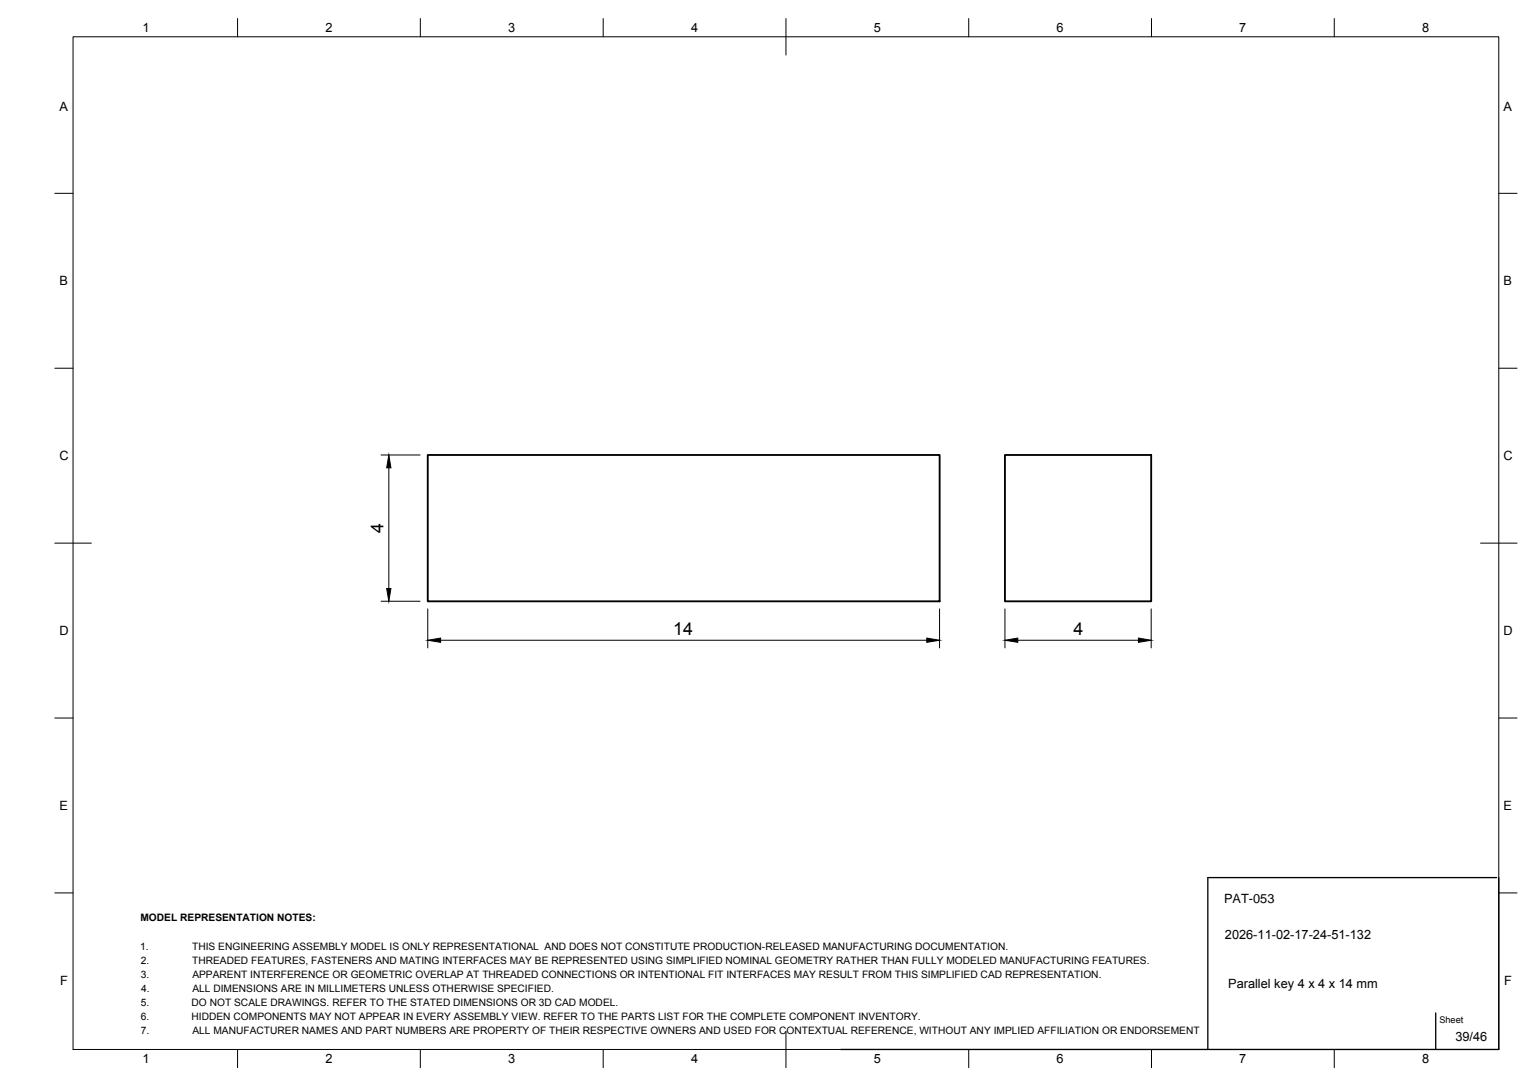
ISO-10303-21;
HEADER;
/* Generated by software containing ST-Developer
 * from STEP Tools, Inc. (www.steptools.com) 
 */

FILE_DESCRIPTION(
/* description */ ('Hand-operated arbor press'),
/* implementation_level */ '2;1');

FILE_NAME(
/* name */ 'Parallel key 4 x 4 x 14 mm.step',
/* time_stamp */ '2026-10-28T03:25:25-07:00',
/* author */ (''),
/* organization */ (''),
/* preprocessor_version */ 'ST-DEVELOPER v20.2',
/* originating_system */ 'Autodesk Translation Framework v15.17.0.0',
/* authorisation */ '');

FILE_SCHEMA (('AUTOMOTIVE_DESIGN { 1 0 10303 214 3 1 1 }'));
ENDSEC;

DATA;
#10=MECHANICAL_DESIGN_GEOMETRIC_PRESENTATION_REPRESENTATION('',(#624),#32751);
#533=SHAPE_REPRESENTATION_RELATIONSHIP('SRR','None',#32965,#575);
#575=ADVANCED_BREP_SHAPE_REPRESENTATION('',(#671),#32739);
#624=STYLED_ITEM('',(#33242),#671);
#671=MANIFOLD_SOLID_BREP('Body1',#12523);
#1214=PLANE('',#13859);
#1215=PLANE('',#13860);
#1216=PLANE('',#13861);
#1217=PLANE('',#13862);
#1218=PLANE('',#13863);
#1219=PLANE('',#13864);
#1807=FACE_OUTER_BOUND('',#2637,.T.);
#1808=FACE_OUTER_BOUND('',#2638,.T.);
#1809=FACE_OUTER_BOUND('',#2639,.T.);
#1810=FACE_OUTER_BOUND('',#2640,.T.);
#1811=FACE_OUTER_BOUND('',#2641,.T.);
#1812=FACE_OUTER_BOUND('',#2642,.T.);
#2637=EDGE_LOOP('',(#10836,#10837,#10838,#10839));
#2638=EDGE_LOOP('',(#10840,#10841,#10842,#10843));
#2639=EDGE_LOOP('',(#10844,#10845,#10846,#10847));
#2640=EDGE_LOOP('',(#10848,#10849,#10850,#10851));
#2641=EDGE_LOOP('',(#10852,#10853,#10854,#10855));
#2642=EDGE_LOOP('',(#10856,#10857,#10858,#10859));
#3762=LINE('',#20662,#4933);
#3763=LINE('',#20664,#4934);
#3764=LINE('',#20666,#4935);
#3765=LINE('',#20667,#4936);
#3766=LINE('',#20670,#4937);
#3767=LINE('',#20672,#4938);
#3768=LINE('',#20673,#4939);
#3769=LINE('',#20676,#4940);
#3770=LINE('',#20678,#4941);
#3771=LINE('',#20679,#4942);
#3772=LINE('',#20681,#4943);
#3773=LINE('',#20682,#4944);
#4933=VECTOR('',#16815,1.);
#4934=VECTOR('',#16816,1.);
#4935=VECTOR('',#16817,1.);
#4936=VECTOR('',#16818,1.);
#4937=VECTOR('',#16821,1.);
#4938=VECTOR('',#16822,1.);
#4939=VECTOR('',#16823,1.);
#4940=VECTOR('',#16826,1.);
#4941=VECTOR('',#16827,1.);
#4942=VECTOR('',#16828,1.);
#4943=VECTOR('',#16831,1.);
#4944=VECTOR('',#16832,1.);
#6399=VERTEX_POINT('',#20660);
#6400=VERTEX_POINT('',#20661);
#6401=VERTEX_POINT('',#20663);
#6402=VERTEX_POINT('',#20665);
#6403=VERTEX_POINT('',#20669);
#6404=VERTEX_POINT('',#20671);
#6405=VERTEX_POINT('',#20675);
#6406=VERTEX_POINT('',#20677);
#7921=EDGE_CURVE('',#6399,#6400,#3762,.T.);
#7922=EDGE_CURVE('',#6400,#6401,#3763,.T.);
#7923=EDGE_CURVE('',#6402,#6401,#3764,.T.);
#7924=EDGE_CURVE('',#6399,#6402,#3765,.T.);
#7925=EDGE_CURVE('',#6403,#6399,#3766,.T.);
#7926=EDGE_CURVE('',#6404,#6402,#3767,.T.);
#7927=EDGE_CURVE('',#6403,#6404,#3768,.T.);
#7928=EDGE_CURVE('',#6405,#6403,#3769,.T.);
#7929=EDGE_CURVE('',#6406,#6404,#3770,.T.);
#7930=EDGE_CURVE('',#6405,#6406,#3771,.T.);
#7931=EDGE_CURVE('',#6400,#6405,#3772,.T.);
#7932=EDGE_CURVE('',#6401,#6406,#3773,.T.);
#10836=ORIENTED_EDGE('',*,*,#7921,.T.);
#10837=ORIENTED_EDGE('',*,*,#7922,.T.);
#10838=ORIENTED_EDGE('',*,*,#7923,.F.);
#10839=ORIENTED_EDGE('',*,*,#7924,.F.);
#10840=ORIENTED_EDGE('',*,*,#7925,.T.);
#10841=ORIENTED_EDGE('',*,*,#7924,.T.);
#10842=ORIENTED_EDGE('',*,*,#7926,.F.);
#10843=ORIENTED_EDGE('',*,*,#7927,.F.);
#10844=ORIENTED_EDGE('',*,*,#7928,.T.);
#10845=ORIENTED_EDGE('',*,*,#7927,.T.);
#10846=ORIENTED_EDGE('',*,*,#7929,.F.);
#10847=ORIENTED_EDGE('',*,*,#7930,.F.);
#10848=ORIENTED_EDGE('',*,*,#7931,.T.);
#10849=ORIENTED_EDGE('',*,*,#7930,.T.);
#10850=ORIENTED_EDGE('',*,*,#7932,.F.);
#10851=ORIENTED_EDGE('',*,*,#7922,.F.);
#10852=ORIENTED_EDGE('',*,*,#7932,.T.);
#10853=ORIENTED_EDGE('',*,*,#7929,.T.);
#10854=ORIENTED_EDGE('',*,*,#7926,.T.);
#10855=ORIENTED_EDGE('',*,*,#7923,.T.);
#10856=ORIENTED_EDGE('',*,*,#7931,.F.);
#10857=ORIENTED_EDGE('',*,*,#7921,.F.);
#10858=ORIENTED_EDGE('',*,*,#7925,.F.);
#10859=ORIENTED_EDGE('',*,*,#7928,.F.);
#12316=ADVANCED_FACE('',(#1807),#1214,.T.);
#12317=ADVANCED_FACE('',(#1808),#1215,.T.);
#12318=ADVANCED_FACE('',(#1809),#1216,.T.);
#12319=ADVANCED_FACE('',(#1810),#1217,.T.);
#12320=ADVANCED_FACE('',(#1811),#1218,.T.);
#12321=ADVANCED_FACE('',(#1812),#1219,.F.);
#12523=CLOSED_SHELL('',(#12316,#12317,#12318,#12319,#12320,#12321));
#13858=AXIS2_PLACEMENT_3D('',#20658,#16811,#16812);
#13859=AXIS2_PLACEMENT_3D('',#20659,#16813,#16814);
#13860=AXIS2_PLACEMENT_3D('',#20668,#16819,#16820);
#13861=AXIS2_PLACEMENT_3D('',#20674,#16824,#16825);
#13862=AXIS2_PLACEMENT_3D('',#20680,#16829,#16830);
#13863=AXIS2_PLACEMENT_3D('',#20683,#16833,#16834);
#13864=AXIS2_PLACEMENT_3D('',#20684,#16835,#16836);
#16811=DIRECTION('axis',(0.,0.,1.));
#16812=DIRECTION('refdir',(1.,0.,0.));
#16813=DIRECTION('center_axis',(0.,1.,0.));
#16814=DIRECTION('ref_axis',(-1.,0.,0.));
#16815=DIRECTION('',(-1.,0.,0.));
#16816=DIRECTION('',(0.,0.,1.));
#16817=DIRECTION('',(-1.,0.,0.));
#16818=DIRECTION('',(0.,0.,1.));
#16819=DIRECTION('center_axis',(1.,0.,0.));
#16820=DIRECTION('ref_axis',(0.,1.,0.));
#16821=DIRECTION('',(0.,1.,0.));
#16822=DIRECTION('',(0.,1.,0.));
#16823=DIRECTION('',(0.,0.,1.));
#16824=DIRECTION('center_axis',(0.,-1.,0.));
#16825=DIRECTION('ref_axis',(1.,0.,0.));
#16826=DIRECTION('',(1.,0.,0.));
#16827=DIRECTION('',(1.,0.,0.));
#16828=DIRECTION('',(0.,0.,1.));
#16829=DIRECTION('center_axis',(-1.,0.,0.));
#16830=DIRECTION('ref_axis',(0.,-1.,0.));
#16831=DIRECTION('',(0.,-1.,0.));
#16832=DIRECTION('',(0.,-1.,0.));
#16833=DIRECTION('center_axis',(0.,0.,1.));
#16834=DIRECTION('ref_axis',(1.,0.,0.));
#16835=DIRECTION('center_axis',(0.,0.,1.));
#16836=DIRECTION('ref_axis',(1.,0.,0.));
#20658=CARTESIAN_POINT('',(0.,0.,0.));
#20659=CARTESIAN_POINT('Origin',(-2.5,1.2,19.8));
#20660=CARTESIAN_POINT('',(-2.5,1.2,19.8));
#20661=CARTESIAN_POINT('',(-2.9,1.2,19.8));
#20662=CARTESIAN_POINT('',(-2.5,1.2,19.8));
#20663=CARTESIAN_POINT('',(-2.9,1.2,20.2));
#20664=CARTESIAN_POINT('',(-2.9,1.2,19.8));
#20665=CARTESIAN_POINT('',(-2.5,1.2,20.2));
#20666=CARTESIAN_POINT('',(-2.5,1.2,20.2));
#20667=CARTESIAN_POINT('',(-2.5,1.2,19.8));
#20668=CARTESIAN_POINT('Origin',(-2.5,-0.2,19.8));
#20669=CARTESIAN_POINT('',(-2.5,-0.2,19.8));
#20670=CARTESIAN_POINT('',(-2.5,-0.2,19.8));
#20671=CARTESIAN_POINT('',(-2.5,-0.2,20.2));
#20672=CARTESIAN_POINT('',(-2.5,-0.2,20.2));
#20673=CARTESIAN_POINT('',(-2.5,-0.2,19.8));
#20674=CARTESIAN_POINT('Origin',(-2.9,-0.2,19.8));
#20675=CARTESIAN_POINT('',(-2.9,-0.2,19.8));
#20676=CARTESIAN_POINT('',(-2.9,-0.2,19.8));
#20677=CARTESIAN_POINT('',(-2.9,-0.2,20.2));
#20678=CARTESIAN_POINT('',(-2.9,-0.2,20.2));
#20679=CARTESIAN_POINT('',(-2.9,-0.2,19.8));
#20680=CARTESIAN_POINT('Origin',(-2.9,1.2,19.8));
#20681=CARTESIAN_POINT('',(-2.9,1.2,19.8));
#20682=CARTESIAN_POINT('',(-2.9,1.2,20.2));
#20683=CARTESIAN_POINT('Origin',(-2.7,0.5,20.2));
#20684=CARTESIAN_POINT('Origin',(-2.7,0.5,19.8));
#32690=UNCERTAINTY_MEASURE_WITH_UNIT(LENGTH_MEASURE(0.001),#32752,
'DISTANCE_ACCURACY_VALUE',
'Maximum model space distance between geometric entities at asserted c
onnectivities');
#32702=UNCERTAINTY_MEASURE_WITH_UNIT(LENGTH_MEASURE(0.001),#32752,
'DISTANCE_ACCURACY_VALUE',
'Maximum model space distance between geometric entities at asserted c
onnectivities');
#32739=(
GEOMETRIC_REPRESENTATION_CONTEXT(3)
GLOBAL_UNCERTAINTY_ASSIGNED_CONTEXT((#32690))
GLOBAL_UNIT_ASSIGNED_CONTEXT((#32752,#32754,#32755))
REPRESENTATION_CONTEXT('','3D')
);
#32751=(
GEOMETRIC_REPRESENTATION_CONTEXT(3)
GLOBAL_UNCERTAINTY_ASSIGNED_CONTEXT((#32702))
GLOBAL_UNIT_ASSIGNED_CONTEXT((#32752,#32754,#32755))
REPRESENTATION_CONTEXT('','3D')
);
#32752=(
LENGTH_UNIT()
NAMED_UNIT(*)
SI_UNIT(.CENTI.,.METRE.)
);
#32754=(
NAMED_UNIT(*)
PLANE_ANGLE_UNIT()
SI_UNIT($,.RADIAN.)
);
#32755=(
NAMED_UNIT(*)
SI_UNIT($,.STERADIAN.)
SOLID_ANGLE_UNIT()
);
#32792=SHAPE_DEFINITION_REPRESENTATION(#32849,#32965);
#32849=PRODUCT_DEFINITION_SHAPE('',$,#33014);
#32965=SHAPE_REPRESENTATION('',(#13858),#32739);
#32977=PRODUCT_DEFINITION_CONTEXT('part definition',#33123,'design');
#33014=PRODUCT_DEFINITION('Parallel key 4 x 4 x 14 mm',
'Parallel key 4 x 4 x 14 mm',#33062,#32977);
#33062=PRODUCT_DEFINITION_FORMATION('',$,#33161);
#33123=APPLICATION_CONTEXT(
'Core Data for Automotive Mechanical Design Process');
#33124=PRODUCT_CONTEXT('part definition',#33123,'mechanical');
#33161=PRODUCT('Parallel key 4 x 4 x 14 mm',
'Parallel key 4 x 4 x 14 mm','Parallel key 4 x 4 x 14 mm',(#33124));
#33236=COLOUR_RGB('Grey',0.48,0.52,0.57);
#33237=FILL_AREA_STYLE_COLOUR('',#33236);
#33238=FILL_AREA_STYLE('',(#33237));
#33239=SURFACE_STYLE_FILL_AREA(#33238);
#33240=SURFACE_SIDE_STYLE('',(#33239));
#33241=SURFACE_STYLE_USAGE(.BOTH.,#33240);
#33242=PRESENTATION_STYLE_ASSIGNMENT((#33241));
ENDSEC;
END-ISO-10303-21;
